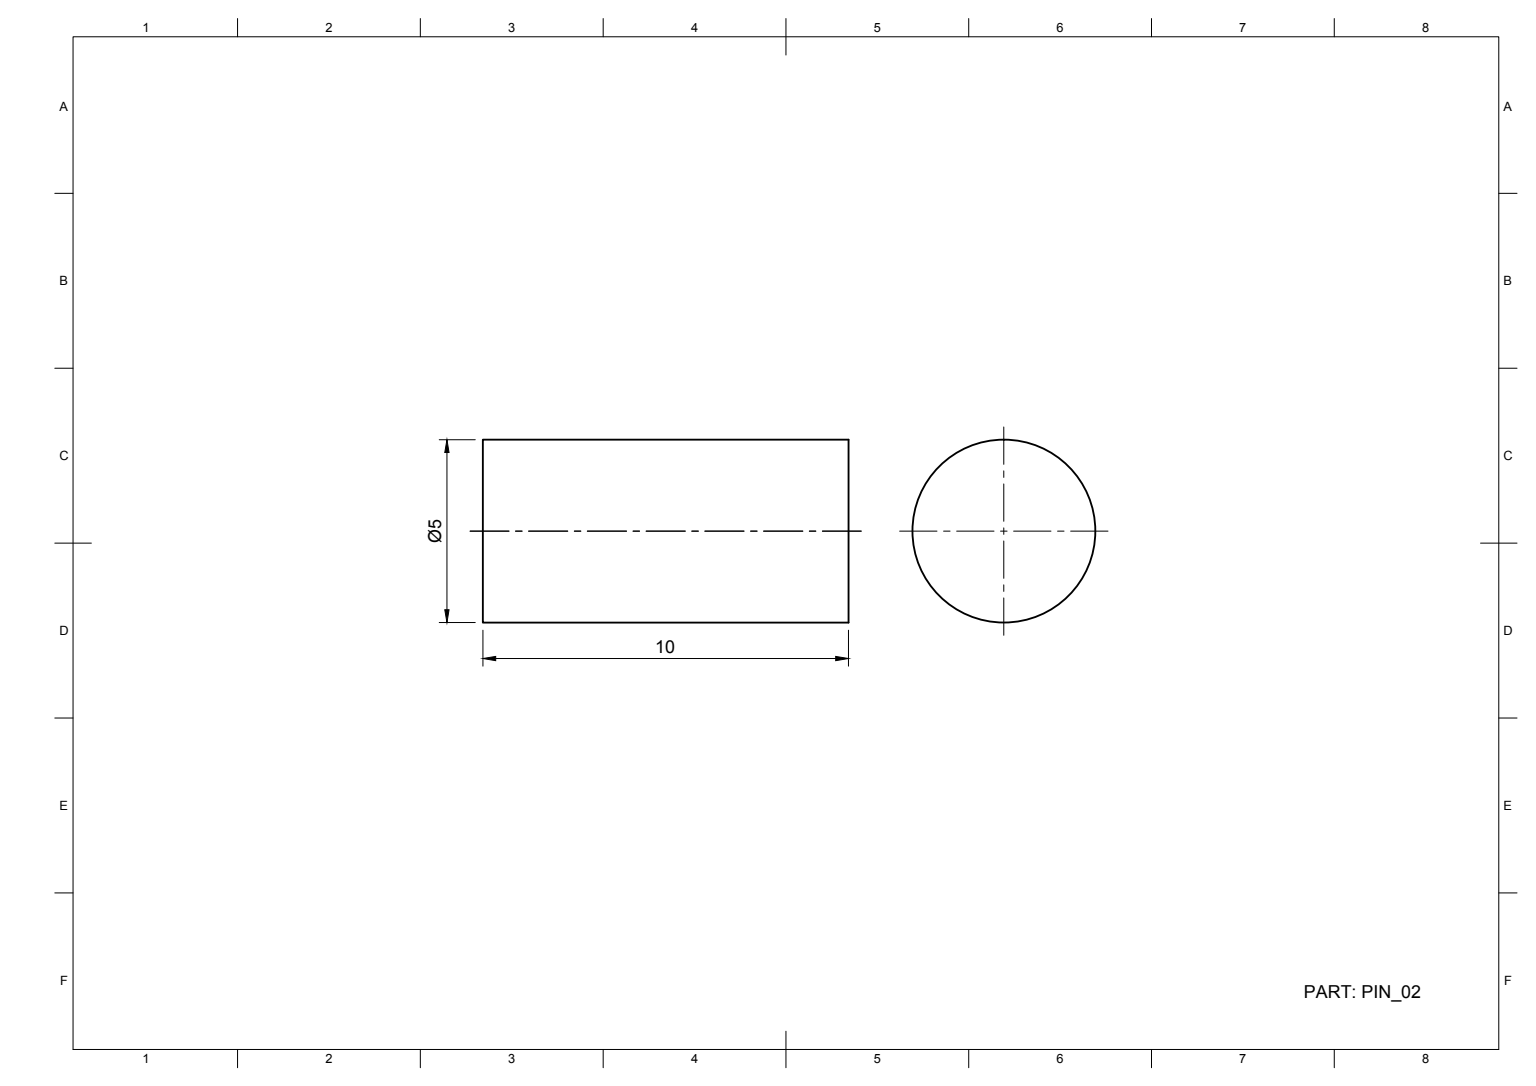
ISO-10303-21;
HEADER;
/* Generated by software containing ST-Developer
 * from STEP Tools, Inc. (www.steptools.com) 
 */

FILE_DESCRIPTION(
/* description */ (''),
/* implementation_level */ '2;1');

FILE_NAME(
/* name */ 'Pin_02.step',
/* time_stamp */ '2026-09-20T21:52:48+06:00',
/* author */ (''),
/* organization */ (''),
/* preprocessor_version */ 'ST-DEVELOPER v20.2',
/* originating_system */ 'Autodesk Translation Framework v15.15.0.0',
/* authorisation */ '');

FILE_SCHEMA (('AUTOMOTIVE_DESIGN { 1 0 10303 214 3 1 1 }'));
ENDSEC;

DATA;
#10=MECHANICAL_DESIGN_GEOMETRIC_PRESENTATION_REPRESENTATION('',(#61),#2203);
#45=SHAPE_REPRESENTATION_RELATIONSHIP('SRR','None',#2237,#53);
#53=ADVANCED_BREP_SHAPE_REPRESENTATION('',(#69),#2197);
#61=STYLED_ITEM('',(#2286),#69);
#69=MANIFOLD_SOLID_BREP('Pin_02',#1228);
#109=CIRCLE('',#1378,2.5);
#110=CIRCLE('',#1380,2.5);
#147=CYLINDRICAL_SURFACE('',#1379,2.5);
#191=FACE_OUTER_BOUND('',#262,.T.);
#192=FACE_OUTER_BOUND('',#263,.T.);
#193=FACE_OUTER_BOUND('',#264,.T.);
#262=EDGE_LOOP('',(#952));
#263=EDGE_LOOP('',(#953,#954,#955,#956));
#264=EDGE_LOOP('',(#957));
#371=LINE('',#2004,#481);
#481=VECTOR('',#1629,2.5);
#585=VERTEX_POINT('',#2000);
#586=VERTEX_POINT('',#2003);
#716=EDGE_CURVE('',#585,#585,#109,.T.);
#717=EDGE_CURVE('',#585,#586,#371,.T.);
#718=EDGE_CURVE('',#586,#586,#110,.T.);
#952=ORIENTED_EDGE('',*,*,#716,.T.);
#953=ORIENTED_EDGE('',*,*,#716,.F.);
#954=ORIENTED_EDGE('',*,*,#717,.T.);
#955=ORIENTED_EDGE('',*,*,#718,.T.);
#956=ORIENTED_EDGE('',*,*,#717,.F.);
#957=ORIENTED_EDGE('',*,*,#718,.F.);
#1132=PLANE('',#1377);
#1133=PLANE('',#1381);
#1187=ADVANCED_FACE('',(#191),#1132,.T.);
#1188=ADVANCED_FACE('',(#192),#147,.T.);
#1189=ADVANCED_FACE('',(#193),#1133,.T.);
#1228=CLOSED_SHELL('',(#1187,#1188,#1189));
#1376=AXIS2_PLACEMENT_3D('',#1998,#1621,#1622);
#1377=AXIS2_PLACEMENT_3D('',#1999,#1623,#1624);
#1378=AXIS2_PLACEMENT_3D('',#2001,#1625,#1626);
#1379=AXIS2_PLACEMENT_3D('',#2002,#1627,#1628);
#1380=AXIS2_PLACEMENT_3D('',#2005,#1630,#1631);
#1381=AXIS2_PLACEMENT_3D('',#2006,#1632,#1633);
#1621=DIRECTION('axis',(0.,0.,1.));
#1622=DIRECTION('refdir',(1.,0.,0.));
#1623=DIRECTION('center_axis',(0.,-1.,0.));
#1624=DIRECTION('ref_axis',(1.,0.,0.));
#1625=DIRECTION('center_axis',(0.,-1.,0.));
#1626=DIRECTION('ref_axis',(1.,0.,0.));
#1627=DIRECTION('center_axis',(0.,-1.,0.));
#1628=DIRECTION('ref_axis',(1.,0.,0.));
#1629=DIRECTION('',(0.,1.,0.));
#1630=DIRECTION('center_axis',(0.,-1.,0.));
#1631=DIRECTION('ref_axis',(1.,0.,0.));
#1632=DIRECTION('center_axis',(0.,1.,0.));
#1633=DIRECTION('ref_axis',(0.,0.,1.));
#1998=CARTESIAN_POINT('',(0.,0.,0.));
#1999=CARTESIAN_POINT('Origin',(1.66533453693773E-15,-5.,72.8759738016714));
#2000=CARTESIAN_POINT('',(-2.5,-5.,72.8759738016714));
#2001=CARTESIAN_POINT('Origin',(1.53080849893419E-15,-5.,72.8759738016714));
#2002=CARTESIAN_POINT('Origin',(1.53080849893419E-15,3.,72.8759738016714));
#2003=CARTESIAN_POINT('',(-2.5,5.,72.8759738016714));
#2004=CARTESIAN_POINT('',(-2.5,3.,72.8759738016714));
#2005=CARTESIAN_POINT('Origin',(1.53080849893419E-15,5.,72.8759738016714));
#2006=CARTESIAN_POINT('Origin',(0.,5.,50.));
#2187=UNCERTAINTY_MEASURE_WITH_UNIT(LENGTH_MEASURE(0.01),#2204,
'DISTANCE_ACCURACY_VALUE',
'Maximum model space distance between geometric entities at asserted c
onnectivities');
#2193=UNCERTAINTY_MEASURE_WITH_UNIT(LENGTH_MEASURE(0.01),#2204,
'DISTANCE_ACCURACY_VALUE',
'Maximum model space distance between geometric entities at asserted c
onnectivities');
#2197=(
GEOMETRIC_REPRESENTATION_CONTEXT(3)
GLOBAL_UNCERTAINTY_ASSIGNED_CONTEXT((#2187))
GLOBAL_UNIT_ASSIGNED_CONTEXT((#2204,#2206,#2207))
REPRESENTATION_CONTEXT('','3D')
);
#2203=(
GEOMETRIC_REPRESENTATION_CONTEXT(3)
GLOBAL_UNCERTAINTY_ASSIGNED_CONTEXT((#2193))
GLOBAL_UNIT_ASSIGNED_CONTEXT((#2204,#2206,#2207))
REPRESENTATION_CONTEXT('','3D')
);
#2204=(
LENGTH_UNIT()
NAMED_UNIT(*)
SI_UNIT(.MILLI.,.METRE.)
);
#2206=(
NAMED_UNIT(*)
PLANE_ANGLE_UNIT()
SI_UNIT($,.RADIAN.)
);
#2207=(
NAMED_UNIT(*)
SI_UNIT($,.STERADIAN.)
SOLID_ANGLE_UNIT()
);
#2211=SHAPE_DEFINITION_REPRESENTATION(#2220,#2237);
#2220=PRODUCT_DEFINITION_SHAPE('',$,#2247);
#2237=SHAPE_REPRESENTATION('',(#1376),#2197);
#2243=PRODUCT_DEFINITION_CONTEXT('part definition',#2272,'design');
#2247=PRODUCT_DEFINITION('Pin_02','Pin_02',#2256,#2243);
#2256=PRODUCT_DEFINITION_FORMATION('',$,#2277);
#2272=APPLICATION_CONTEXT(
'Core Data for Automotive Mechanical Design Process');
#2273=PRODUCT_CONTEXT('part definition',#2272,'mechanical');
#2277=PRODUCT('Pin_02','Pin_02',$,(#2273));
#2286=PRESENTATION_STYLE_ASSIGNMENT((#2290));
#2290=SURFACE_STYLE_USAGE(.BOTH.,#2294);
#2294=SURFACE_SIDE_STYLE('',(#2298));
#2298=SURFACE_STYLE_FILL_AREA(#2302);
#2302=FILL_AREA_STYLE('Surface - Matte',(#2306));
#2306=FILL_AREA_STYLE_COLOUR('Surface - Matte',#2310);
#2310=COLOUR_RGB('Surface - Matte', 0.31764706, 0.68627451, 0.89019608);
ENDSEC;
END-ISO-10303-21;
